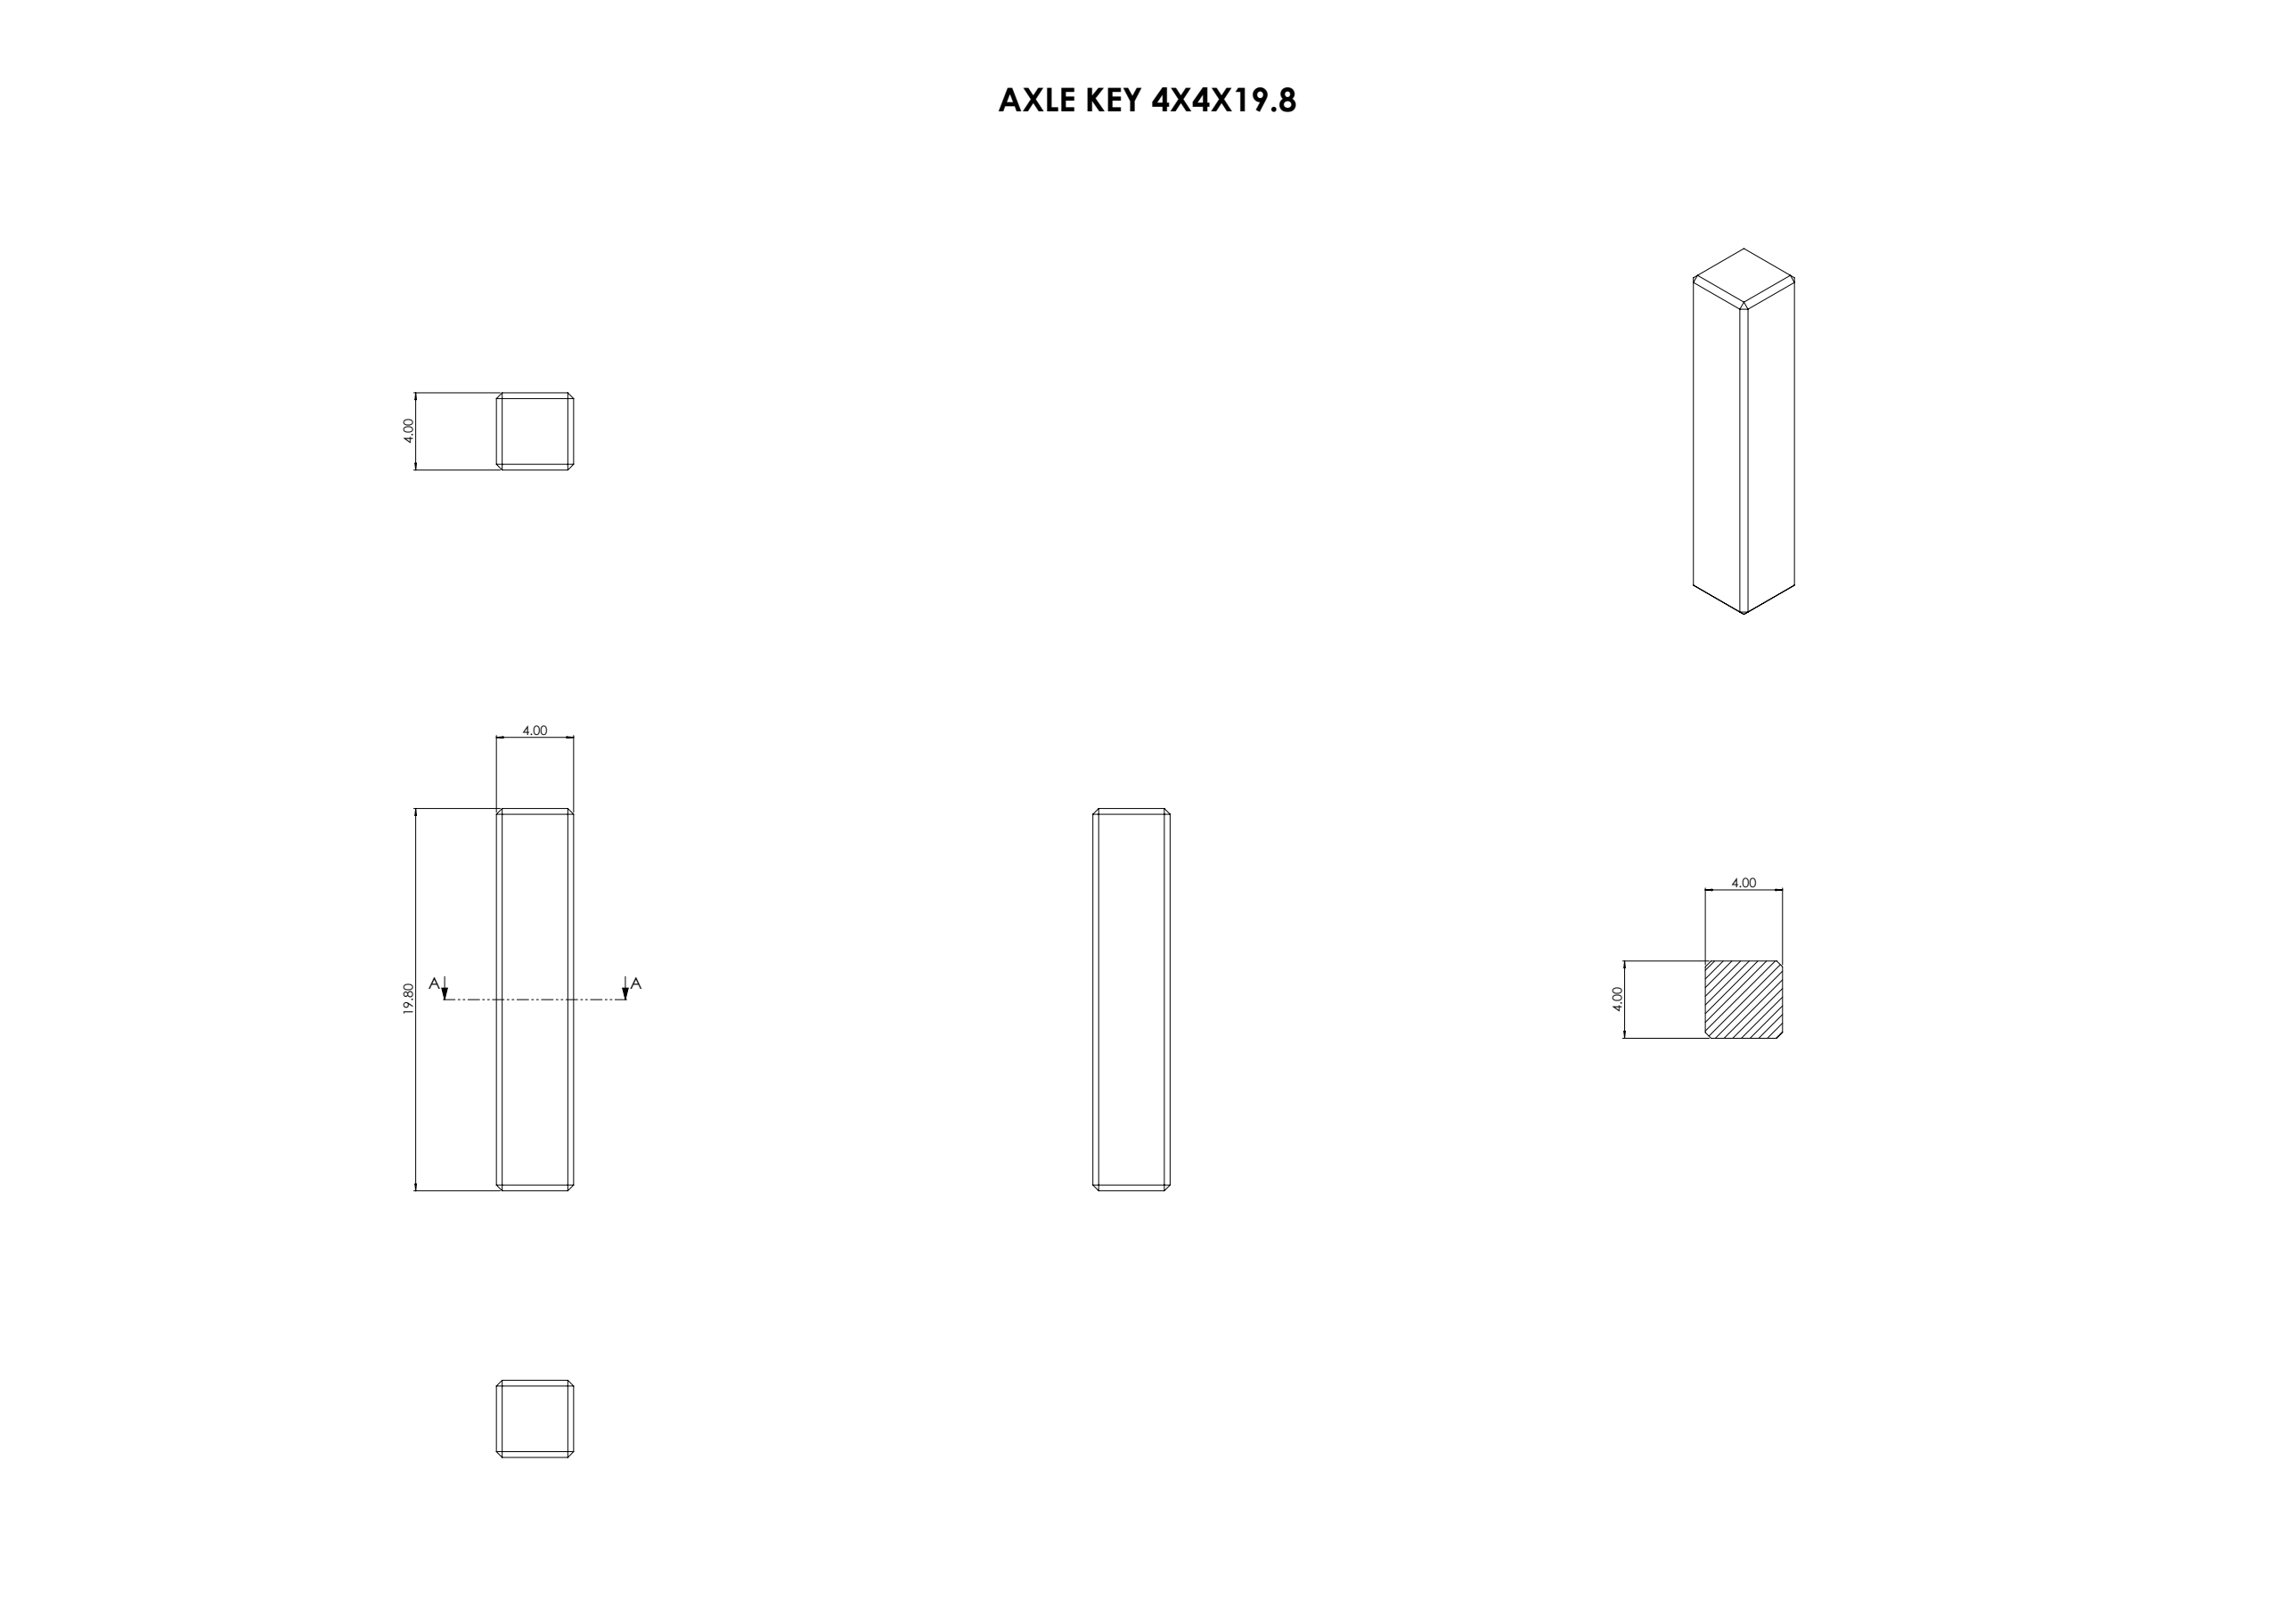
ISO-10303-21;
HEADER;
/* Generated by software containing ST-Developer
 * from STEP Tools, Inc. (www.steptools.com) 
 */

FILE_DESCRIPTION(
/* description */ (''),
/* implementation_level */ '2;1');

FILE_NAME(
/* name */ '09_Axle_Key_4x4x19.8.step',
/* time_stamp */ '2026-10-11T13:00:10-07:00',
/* author */ (''),
/* organization */ (''),
/* preprocessor_version */ 'ST-DEVELOPER v20.2',
/* originating_system */ 'Autodesk Translation Framework v15.15.0.0',
/* authorisation */ '');

FILE_SCHEMA (('AUTOMOTIVE_DESIGN { 1 0 10303 214 3 1 1 }'));
ENDSEC;

DATA;
#10=MECHANICAL_DESIGN_GEOMETRIC_PRESENTATION_REPRESENTATION('',(#366),#65563);
#344=SHAPE_REPRESENTATION_RELATIONSHIP('SRR','None',#65622,#355);
#355=ADVANCED_BREP_SHAPE_REPRESENTATION('',(#377),#65560);
#366=STYLED_ITEM('',(#65788),#377);
#377=MANIFOLD_SOLID_BREP('Body1',#20016);
#1012=PLANE('',#22010);
#1013=PLANE('',#22011);
#1014=PLANE('',#22012);
#1015=PLANE('',#22013);
#1016=PLANE('',#22014);
#1017=PLANE('',#22015);
#1018=PLANE('',#22016);
#1019=PLANE('',#22017);
#1020=PLANE('',#22018);
#1021=PLANE('',#22019);
#1022=PLANE('',#22020);
#1023=PLANE('',#22021);
#1024=PLANE('',#22022);
#1025=PLANE('',#22023);
#1026=PLANE('',#22024);
#1027=PLANE('',#22025);
#1028=PLANE('',#22026);
#1029=PLANE('',#22027);
#1030=PLANE('',#22028);
#1031=PLANE('',#22029);
#1032=PLANE('',#22030);
#1033=PLANE('',#22031);
#1034=PLANE('',#22032);
#1035=PLANE('',#22033);
#1036=PLANE('',#22034);
#1037=PLANE('',#22035);
#2122=FACE_OUTER_BOUND('',#3350,.T.);
#2123=FACE_OUTER_BOUND('',#3351,.T.);
#2124=FACE_OUTER_BOUND('',#3352,.T.);
#2125=FACE_OUTER_BOUND('',#3353,.T.);
#2126=FACE_OUTER_BOUND('',#3354,.T.);
#2127=FACE_OUTER_BOUND('',#3355,.T.);
#2128=FACE_OUTER_BOUND('',#3356,.T.);
#2129=FACE_OUTER_BOUND('',#3357,.T.);
#2130=FACE_OUTER_BOUND('',#3358,.T.);
#2131=FACE_OUTER_BOUND('',#3359,.T.);
#2132=FACE_OUTER_BOUND('',#3360,.T.);
#2133=FACE_OUTER_BOUND('',#3361,.T.);
#2134=FACE_OUTER_BOUND('',#3362,.T.);
#2135=FACE_OUTER_BOUND('',#3363,.T.);
#2136=FACE_OUTER_BOUND('',#3364,.T.);
#2137=FACE_OUTER_BOUND('',#3365,.T.);
#2138=FACE_OUTER_BOUND('',#3366,.T.);
#2139=FACE_OUTER_BOUND('',#3367,.T.);
#2140=FACE_OUTER_BOUND('',#3368,.T.);
#2141=FACE_OUTER_BOUND('',#3369,.T.);
#2142=FACE_OUTER_BOUND('',#3370,.T.);
#2143=FACE_OUTER_BOUND('',#3371,.T.);
#2144=FACE_OUTER_BOUND('',#3372,.T.);
#2145=FACE_OUTER_BOUND('',#3373,.T.);
#2146=FACE_OUTER_BOUND('',#3374,.T.);
#2147=FACE_OUTER_BOUND('',#3375,.T.);
#3350=EDGE_LOOP('',(#17338,#17339,#17340));
#3351=EDGE_LOOP('',(#17341,#17342,#17343));
#3352=EDGE_LOOP('',(#17344,#17345,#17346));
#3353=EDGE_LOOP('',(#17347,#17348,#17349));
#3354=EDGE_LOOP('',(#17350,#17351,#17352,#17353));
#3355=EDGE_LOOP('',(#17354,#17355,#17356));
#3356=EDGE_LOOP('',(#17357,#17358,#17359));
#3357=EDGE_LOOP('',(#17360,#17361,#17362,#17363));
#3358=EDGE_LOOP('',(#17364,#17365,#17366));
#3359=EDGE_LOOP('',(#17367,#17368,#17369,#17370));
#3360=EDGE_LOOP('',(#17371,#17372,#17373,#17374));
#3361=EDGE_LOOP('',(#17375,#17376,#17377));
#3362=EDGE_LOOP('',(#17378,#17379,#17380,#17381));
#3363=EDGE_LOOP('',(#17382,#17383,#17384,#17385));
#3364=EDGE_LOOP('',(#17386,#17387,#17388,#17389));
#3365=EDGE_LOOP('',(#17390,#17391,#17392,#17393));
#3366=EDGE_LOOP('',(#17394,#17395,#17396,#17397));
#3367=EDGE_LOOP('',(#17398,#17399,#17400,#17401));
#3368=EDGE_LOOP('',(#17402,#17403,#17404,#17405));
#3369=EDGE_LOOP('',(#17406,#17407,#17408,#17409));
#3370=EDGE_LOOP('',(#17410,#17411,#17412,#17413));
#3371=EDGE_LOOP('',(#17414,#17415,#17416,#17417));
#3372=EDGE_LOOP('',(#17418,#17419,#17420,#17421));
#3373=EDGE_LOOP('',(#17422,#17423,#17424,#17425));
#3374=EDGE_LOOP('',(#17426,#17427,#17428,#17429));
#3375=EDGE_LOOP('',(#17430,#17431,#17432,#17433));
#6130=LINE('',#62589,#7022);
#6131=LINE('',#62591,#7023);
#6132=LINE('',#62592,#7024);
#6133=LINE('',#62596,#7025);
#6134=LINE('',#62598,#7026);
#6135=LINE('',#62599,#7027);
#6136=LINE('',#62603,#7028);
#6137=LINE('',#62605,#7029);
#6138=LINE('',#62606,#7030);
#6139=LINE('',#62610,#7031);
#6140=LINE('',#62612,#7032);
#6141=LINE('',#62613,#7033);
#6142=LINE('',#62615,#7034);
#6143=LINE('',#62616,#7035);
#6144=LINE('',#62620,#7036);
#6145=LINE('',#62622,#7037);
#6146=LINE('',#62623,#7038);
#6147=LINE('',#62627,#7039);
#6148=LINE('',#62629,#7040);
#6149=LINE('',#62630,#7041);
#6150=LINE('',#62632,#7042);
#6151=LINE('',#62633,#7043);
#6152=LINE('',#62637,#7044);
#6153=LINE('',#62639,#7045);
#6154=LINE('',#62640,#7046);
#6155=LINE('',#62642,#7047);
#6156=LINE('',#62643,#7048);
#6157=LINE('',#62645,#7049);
#6158=LINE('',#62646,#7050);
#6159=LINE('',#62650,#7051);
#6160=LINE('',#62652,#7052);
#6161=LINE('',#62653,#7053);
#6162=LINE('',#62655,#7054);
#6163=LINE('',#62656,#7055);
#6164=LINE('',#62658,#7056);
#6165=LINE('',#62659,#7057);
#6166=LINE('',#62661,#7058);
#6167=LINE('',#62662,#7059);
#6168=LINE('',#62664,#7060);
#6169=LINE('',#62665,#7061);
#6170=LINE('',#62667,#7062);
#6171=LINE('',#62668,#7063);
#6172=LINE('',#62670,#7064);
#6173=LINE('',#62671,#7065);
#6174=LINE('',#62673,#7066);
#6175=LINE('',#62674,#7067);
#6176=LINE('',#62676,#7068);
#6177=LINE('',#62677,#7069);
#7022=VECTOR('',#26831,10.);
#7023=VECTOR('',#26832,10.);
#7024=VECTOR('',#26833,10.);
#7025=VECTOR('',#26836,10.);
#7026=VECTOR('',#26837,10.);
#7027=VECTOR('',#26838,10.);
#7028=VECTOR('',#26841,10.);
#7029=VECTOR('',#26842,10.);
#7030=VECTOR('',#26843,10.);
#7031=VECTOR('',#26846,10.);
#7032=VECTOR('',#26847,10.);
#7033=VECTOR('',#26848,10.);
#7034=VECTOR('',#26851,10.);
#7035=VECTOR('',#26852,10.);
#7036=VECTOR('',#26855,10.);
#7037=VECTOR('',#26856,10.);
#7038=VECTOR('',#26857,10.);
#7039=VECTOR('',#26860,10.);
#7040=VECTOR('',#26861,10.);
#7041=VECTOR('',#26862,10.);
#7042=VECTOR('',#26865,10.);
#7043=VECTOR('',#26866,10.);
#7044=VECTOR('',#26869,10.);
#7045=VECTOR('',#26870,10.);
#7046=VECTOR('',#26871,10.);
#7047=VECTOR('',#26874,10.);
#7048=VECTOR('',#26875,10.);
#7049=VECTOR('',#26878,10.);
#7050=VECTOR('',#26879,10.);
#7051=VECTOR('',#26882,10.);
#7052=VECTOR('',#26883,10.);
#7053=VECTOR('',#26884,10.);
#7054=VECTOR('',#26887,10.);
#7055=VECTOR('',#26888,10.);
#7056=VECTOR('',#26891,10.);
#7057=VECTOR('',#26892,10.);
#7058=VECTOR('',#26895,10.);
#7059=VECTOR('',#26896,10.);
#7060=VECTOR('',#26899,10.);
#7061=VECTOR('',#26900,10.);
#7062=VECTOR('',#26903,10.);
#7063=VECTOR('',#26904,10.);
#7064=VECTOR('',#26907,10.);
#7065=VECTOR('',#26908,10.);
#7066=VECTOR('',#26911,10.);
#7067=VECTOR('',#26912,10.);
#7068=VECTOR('',#26915,10.);
#7069=VECTOR('',#26916,10.);
#8833=VERTEX_POINT('',#62587);
#8834=VERTEX_POINT('',#62588);
#8835=VERTEX_POINT('',#62590);
#8836=VERTEX_POINT('',#62594);
#8837=VERTEX_POINT('',#62595);
#8838=VERTEX_POINT('',#62597);
#8839=VERTEX_POINT('',#62601);
#8840=VERTEX_POINT('',#62602);
#8841=VERTEX_POINT('',#62604);
#8842=VERTEX_POINT('',#62608);
#8843=VERTEX_POINT('',#62609);
#8844=VERTEX_POINT('',#62611);
#8845=VERTEX_POINT('',#62618);
#8846=VERTEX_POINT('',#62619);
#8847=VERTEX_POINT('',#62621);
#8848=VERTEX_POINT('',#62625);
#8849=VERTEX_POINT('',#62626);
#8850=VERTEX_POINT('',#62628);
#8851=VERTEX_POINT('',#62635);
#8852=VERTEX_POINT('',#62636);
#8853=VERTEX_POINT('',#62638);
#8854=VERTEX_POINT('',#62648);
#8855=VERTEX_POINT('',#62649);
#8856=VERTEX_POINT('',#62651);
#11702=EDGE_CURVE('',#8833,#8834,#6130,.T.);
#11703=EDGE_CURVE('',#8835,#8833,#6131,.T.);
#11704=EDGE_CURVE('',#8834,#8835,#6132,.T.);
#11705=EDGE_CURVE('',#8836,#8837,#6133,.T.);
#11706=EDGE_CURVE('',#8838,#8836,#6134,.T.);
#11707=EDGE_CURVE('',#8837,#8838,#6135,.T.);
#11708=EDGE_CURVE('',#8839,#8840,#6136,.T.);
#11709=EDGE_CURVE('',#8841,#8839,#6137,.T.);
#11710=EDGE_CURVE('',#8840,#8841,#6138,.T.);
#11711=EDGE_CURVE('',#8842,#8843,#6139,.T.);
#11712=EDGE_CURVE('',#8844,#8842,#6140,.T.);
#11713=EDGE_CURVE('',#8843,#8844,#6141,.T.);
#11714=EDGE_CURVE('',#8833,#8844,#6142,.T.);
#11715=EDGE_CURVE('',#8842,#8835,#6143,.T.);
#11716=EDGE_CURVE('',#8845,#8846,#6144,.T.);
#11717=EDGE_CURVE('',#8847,#8845,#6145,.T.);
#11718=EDGE_CURVE('',#8846,#8847,#6146,.T.);
#11719=EDGE_CURVE('',#8848,#8849,#6147,.T.);
#11720=EDGE_CURVE('',#8850,#8848,#6148,.T.);
#11721=EDGE_CURVE('',#8849,#8850,#6149,.T.);
#11722=EDGE_CURVE('',#8836,#8850,#6150,.T.);
#11723=EDGE_CURVE('',#8848,#8838,#6151,.T.);
#11724=EDGE_CURVE('',#8851,#8852,#6152,.T.);
#11725=EDGE_CURVE('',#8853,#8851,#6153,.T.);
#11726=EDGE_CURVE('',#8852,#8853,#6154,.T.);
#11727=EDGE_CURVE('',#8851,#8841,#6155,.T.);
#11728=EDGE_CURVE('',#8839,#8853,#6156,.T.);
#11729=EDGE_CURVE('',#8843,#8852,#6157,.T.);
#11730=EDGE_CURVE('',#8853,#8842,#6158,.T.);
#11731=EDGE_CURVE('',#8854,#8855,#6159,.T.);
#11732=EDGE_CURVE('',#8856,#8854,#6160,.T.);
#11733=EDGE_CURVE('',#8855,#8856,#6161,.T.);
#11734=EDGE_CURVE('',#8845,#8856,#6162,.T.);
#11735=EDGE_CURVE('',#8854,#8847,#6163,.T.);
#11736=EDGE_CURVE('',#8852,#8855,#6164,.T.);
#11737=EDGE_CURVE('',#8856,#8851,#6165,.T.);
#11738=EDGE_CURVE('',#8855,#8849,#6166,.T.);
#11739=EDGE_CURVE('',#8850,#8854,#6167,.T.);
#11740=EDGE_CURVE('',#8849,#8843,#6168,.T.);
#11741=EDGE_CURVE('',#8844,#8848,#6169,.T.);
#11742=EDGE_CURVE('',#8837,#8846,#6170,.T.);
#11743=EDGE_CURVE('',#8847,#8836,#6171,.T.);
#11744=EDGE_CURVE('',#8846,#8840,#6172,.T.);
#11745=EDGE_CURVE('',#8841,#8845,#6173,.T.);
#11746=EDGE_CURVE('',#8840,#8834,#6174,.T.);
#11747=EDGE_CURVE('',#8835,#8839,#6175,.T.);
#11748=EDGE_CURVE('',#8834,#8837,#6176,.T.);
#11749=EDGE_CURVE('',#8838,#8833,#6177,.T.);
#17338=ORIENTED_EDGE('',*,*,#11702,.F.);
#17339=ORIENTED_EDGE('',*,*,#11703,.F.);
#17340=ORIENTED_EDGE('',*,*,#11704,.F.);
#17341=ORIENTED_EDGE('',*,*,#11705,.F.);
#17342=ORIENTED_EDGE('',*,*,#11706,.F.);
#17343=ORIENTED_EDGE('',*,*,#11707,.F.);
#17344=ORIENTED_EDGE('',*,*,#11708,.F.);
#17345=ORIENTED_EDGE('',*,*,#11709,.F.);
#17346=ORIENTED_EDGE('',*,*,#11710,.F.);
#17347=ORIENTED_EDGE('',*,*,#11711,.F.);
#17348=ORIENTED_EDGE('',*,*,#11712,.F.);
#17349=ORIENTED_EDGE('',*,*,#11713,.F.);
#17350=ORIENTED_EDGE('',*,*,#11703,.T.);
#17351=ORIENTED_EDGE('',*,*,#11714,.T.);
#17352=ORIENTED_EDGE('',*,*,#11712,.T.);
#17353=ORIENTED_EDGE('',*,*,#11715,.T.);
#17354=ORIENTED_EDGE('',*,*,#11716,.F.);
#17355=ORIENTED_EDGE('',*,*,#11717,.F.);
#17356=ORIENTED_EDGE('',*,*,#11718,.F.);
#17357=ORIENTED_EDGE('',*,*,#11719,.F.);
#17358=ORIENTED_EDGE('',*,*,#11720,.F.);
#17359=ORIENTED_EDGE('',*,*,#11721,.F.);
#17360=ORIENTED_EDGE('',*,*,#11706,.T.);
#17361=ORIENTED_EDGE('',*,*,#11722,.T.);
#17362=ORIENTED_EDGE('',*,*,#11720,.T.);
#17363=ORIENTED_EDGE('',*,*,#11723,.T.);
#17364=ORIENTED_EDGE('',*,*,#11724,.F.);
#17365=ORIENTED_EDGE('',*,*,#11725,.F.);
#17366=ORIENTED_EDGE('',*,*,#11726,.F.);
#17367=ORIENTED_EDGE('',*,*,#11725,.T.);
#17368=ORIENTED_EDGE('',*,*,#11727,.T.);
#17369=ORIENTED_EDGE('',*,*,#11709,.T.);
#17370=ORIENTED_EDGE('',*,*,#11728,.T.);
#17371=ORIENTED_EDGE('',*,*,#11711,.T.);
#17372=ORIENTED_EDGE('',*,*,#11729,.T.);
#17373=ORIENTED_EDGE('',*,*,#11726,.T.);
#17374=ORIENTED_EDGE('',*,*,#11730,.T.);
#17375=ORIENTED_EDGE('',*,*,#11731,.F.);
#17376=ORIENTED_EDGE('',*,*,#11732,.F.);
#17377=ORIENTED_EDGE('',*,*,#11733,.F.);
#17378=ORIENTED_EDGE('',*,*,#11717,.T.);
#17379=ORIENTED_EDGE('',*,*,#11734,.T.);
#17380=ORIENTED_EDGE('',*,*,#11732,.T.);
#17381=ORIENTED_EDGE('',*,*,#11735,.T.);
#17382=ORIENTED_EDGE('',*,*,#11724,.T.);
#17383=ORIENTED_EDGE('',*,*,#11736,.T.);
#17384=ORIENTED_EDGE('',*,*,#11733,.T.);
#17385=ORIENTED_EDGE('',*,*,#11737,.T.);
#17386=ORIENTED_EDGE('',*,*,#11731,.T.);
#17387=ORIENTED_EDGE('',*,*,#11738,.T.);
#17388=ORIENTED_EDGE('',*,*,#11721,.T.);
#17389=ORIENTED_EDGE('',*,*,#11739,.T.);
#17390=ORIENTED_EDGE('',*,*,#11719,.T.);
#17391=ORIENTED_EDGE('',*,*,#11740,.T.);
#17392=ORIENTED_EDGE('',*,*,#11713,.T.);
#17393=ORIENTED_EDGE('',*,*,#11741,.T.);
#17394=ORIENTED_EDGE('',*,*,#11705,.T.);
#17395=ORIENTED_EDGE('',*,*,#11742,.T.);
#17396=ORIENTED_EDGE('',*,*,#11718,.T.);
#17397=ORIENTED_EDGE('',*,*,#11743,.T.);
#17398=ORIENTED_EDGE('',*,*,#11716,.T.);
#17399=ORIENTED_EDGE('',*,*,#11744,.T.);
#17400=ORIENTED_EDGE('',*,*,#11710,.T.);
#17401=ORIENTED_EDGE('',*,*,#11745,.T.);
#17402=ORIENTED_EDGE('',*,*,#11708,.T.);
#17403=ORIENTED_EDGE('',*,*,#11746,.T.);
#17404=ORIENTED_EDGE('',*,*,#11704,.T.);
#17405=ORIENTED_EDGE('',*,*,#11747,.T.);
#17406=ORIENTED_EDGE('',*,*,#11702,.T.);
#17407=ORIENTED_EDGE('',*,*,#11748,.T.);
#17408=ORIENTED_EDGE('',*,*,#11707,.T.);
#17409=ORIENTED_EDGE('',*,*,#11749,.T.);
#17410=ORIENTED_EDGE('',*,*,#11723,.F.);
#17411=ORIENTED_EDGE('',*,*,#11741,.F.);
#17412=ORIENTED_EDGE('',*,*,#11714,.F.);
#17413=ORIENTED_EDGE('',*,*,#11749,.F.);
#17414=ORIENTED_EDGE('',*,*,#11728,.F.);
#17415=ORIENTED_EDGE('',*,*,#11747,.F.);
#17416=ORIENTED_EDGE('',*,*,#11715,.F.);
#17417=ORIENTED_EDGE('',*,*,#11730,.F.);
#17418=ORIENTED_EDGE('',*,*,#11729,.F.);
#17419=ORIENTED_EDGE('',*,*,#11740,.F.);
#17420=ORIENTED_EDGE('',*,*,#11738,.F.);
#17421=ORIENTED_EDGE('',*,*,#11736,.F.);
#17422=ORIENTED_EDGE('',*,*,#11735,.F.);
#17423=ORIENTED_EDGE('',*,*,#11739,.F.);
#17424=ORIENTED_EDGE('',*,*,#11722,.F.);
#17425=ORIENTED_EDGE('',*,*,#11743,.F.);
#17426=ORIENTED_EDGE('',*,*,#11734,.F.);
#17427=ORIENTED_EDGE('',*,*,#11745,.F.);
#17428=ORIENTED_EDGE('',*,*,#11727,.F.);
#17429=ORIENTED_EDGE('',*,*,#11737,.F.);
#17430=ORIENTED_EDGE('',*,*,#11742,.F.);
#17431=ORIENTED_EDGE('',*,*,#11748,.F.);
#17432=ORIENTED_EDGE('',*,*,#11746,.F.);
#17433=ORIENTED_EDGE('',*,*,#11744,.F.);
#19818=ADVANCED_FACE('',(#2122),#1012,.T.);
#19819=ADVANCED_FACE('',(#2123),#1013,.T.);
#19820=ADVANCED_FACE('',(#2124),#1014,.T.);
#19821=ADVANCED_FACE('',(#2125),#1015,.T.);
#19822=ADVANCED_FACE('',(#2126),#1016,.T.);
#19823=ADVANCED_FACE('',(#2127),#1017,.T.);
#19824=ADVANCED_FACE('',(#2128),#1018,.T.);
#19825=ADVANCED_FACE('',(#2129),#1019,.T.);
#19826=ADVANCED_FACE('',(#2130),#1020,.T.);
#19827=ADVANCED_FACE('',(#2131),#1021,.T.);
#19828=ADVANCED_FACE('',(#2132),#1022,.T.);
#19829=ADVANCED_FACE('',(#2133),#1023,.T.);
#19830=ADVANCED_FACE('',(#2134),#1024,.T.);
#19831=ADVANCED_FACE('',(#2135),#1025,.T.);
#19832=ADVANCED_FACE('',(#2136),#1026,.T.);
#19833=ADVANCED_FACE('',(#2137),#1027,.T.);
#19834=ADVANCED_FACE('',(#2138),#1028,.T.);
#19835=ADVANCED_FACE('',(#2139),#1029,.T.);
#19836=ADVANCED_FACE('',(#2140),#1030,.T.);
#19837=ADVANCED_FACE('',(#2141),#1031,.T.);
#19838=ADVANCED_FACE('',(#2142),#1032,.T.);
#19839=ADVANCED_FACE('',(#2143),#1033,.T.);
#19840=ADVANCED_FACE('',(#2144),#1034,.T.);
#19841=ADVANCED_FACE('',(#2145),#1035,.T.);
#19842=ADVANCED_FACE('',(#2146),#1036,.T.);
#19843=ADVANCED_FACE('',(#2147),#1037,.T.);
#20016=CLOSED_SHELL('',(#19818,#19819,#19820,#19821,#19822,#19823,#19824,
#19825,#19826,#19827,#19828,#19829,#19830,#19831,#19832,#19833,#19834,#19835,
#19836,#19837,#19838,#19839,#19840,#19841,#19842,#19843));
#22009=AXIS2_PLACEMENT_3D('',#62585,#26827,#26828);
#22010=AXIS2_PLACEMENT_3D('',#62586,#26829,#26830);
#22011=AXIS2_PLACEMENT_3D('',#62593,#26834,#26835);
#22012=AXIS2_PLACEMENT_3D('',#62600,#26839,#26840);
#22013=AXIS2_PLACEMENT_3D('',#62607,#26844,#26845);
#22014=AXIS2_PLACEMENT_3D('',#62614,#26849,#26850);
#22015=AXIS2_PLACEMENT_3D('',#62617,#26853,#26854);
#22016=AXIS2_PLACEMENT_3D('',#62624,#26858,#26859);
#22017=AXIS2_PLACEMENT_3D('',#62631,#26863,#26864);
#22018=AXIS2_PLACEMENT_3D('',#62634,#26867,#26868);
#22019=AXIS2_PLACEMENT_3D('',#62641,#26872,#26873);
#22020=AXIS2_PLACEMENT_3D('',#62644,#26876,#26877);
#22021=AXIS2_PLACEMENT_3D('',#62647,#26880,#26881);
#22022=AXIS2_PLACEMENT_3D('',#62654,#26885,#26886);
#22023=AXIS2_PLACEMENT_3D('',#62657,#26889,#26890);
#22024=AXIS2_PLACEMENT_3D('',#62660,#26893,#26894);
#22025=AXIS2_PLACEMENT_3D('',#62663,#26897,#26898);
#22026=AXIS2_PLACEMENT_3D('',#62666,#26901,#26902);
#22027=AXIS2_PLACEMENT_3D('',#62669,#26905,#26906);
#22028=AXIS2_PLACEMENT_3D('',#62672,#26909,#26910);
#22029=AXIS2_PLACEMENT_3D('',#62675,#26913,#26914);
#22030=AXIS2_PLACEMENT_3D('',#62678,#26917,#26918);
#22031=AXIS2_PLACEMENT_3D('',#62679,#26919,#26920);
#22032=AXIS2_PLACEMENT_3D('',#62680,#26921,#26922);
#22033=AXIS2_PLACEMENT_3D('',#62681,#26923,#26924);
#22034=AXIS2_PLACEMENT_3D('',#62682,#26925,#26926);
#22035=AXIS2_PLACEMENT_3D('',#62683,#26927,#26928);
#26827=DIRECTION('axis',(0.,0.,1.));
#26828=DIRECTION('refdir',(1.,0.,0.));
#26829=DIRECTION('center_axis',(0.577350269189626,0.577350269189626,0.577350269189626));
#26830=DIRECTION('ref_axis',(0.707106781186548,0.,-0.707106781186547));
#26831=DIRECTION('',(-0.707106781186548,0.,0.707106781186547));
#26832=DIRECTION('',(0.707106781186548,-0.707106781186548,0.));
#26833=DIRECTION('',(0.,0.707106781186548,-0.707106781186547));
#26834=DIRECTION('center_axis',(0.577350269189626,-0.577350269189626,0.577350269189626));
#26835=DIRECTION('ref_axis',(0.707106781186548,0.,-0.707106781186547));
#26836=DIRECTION('',(0.,0.707106781186548,0.707106781186547));
#26837=DIRECTION('',(-0.707106781186548,-0.707106781186548,0.));
#26838=DIRECTION('',(0.707106781186548,0.,-0.707106781186547));
#26839=DIRECTION('center_axis',(-0.577350269189626,0.577350269189626,0.577350269189626));
#26840=DIRECTION('ref_axis',(0.707106781186548,0.,0.707106781186547));
#26841=DIRECTION('',(0.,-0.707106781186548,0.707106781186547));
#26842=DIRECTION('',(0.707106781186548,0.707106781186548,0.));
#26843=DIRECTION('',(-0.707106781186548,0.,-0.707106781186547));
#26844=DIRECTION('center_axis',(0.577350269189626,0.577350269189626,-0.577350269189626));
#26845=DIRECTION('ref_axis',(-0.707106781186548,0.,-0.707106781186547));
#26846=DIRECTION('',(0.,-0.707106781186548,-0.707106781186547));
#26847=DIRECTION('',(-0.707106781186548,0.707106781186548,0.));
#26848=DIRECTION('',(0.707106781186548,0.,0.707106781186547));
#26849=DIRECTION('center_axis',(0.707106781186548,0.707106781186548,0.));
#26850=DIRECTION('ref_axis',(0.,0.,-1.));
#26851=DIRECTION('',(0.,0.,-1.));
#26852=DIRECTION('',(0.,0.,1.));
#26853=DIRECTION('center_axis',(-0.577350269189624,-0.577350269189629,0.577350269189625));
#26854=DIRECTION('ref_axis',(0.707106781186548,0.,0.707106781186547));
#26855=DIRECTION('',(0.707106781186548,0.,0.707106781186547));
#26856=DIRECTION('',(-0.70710678118655,0.707106781186545,0.));
#26857=DIRECTION('',(5.23364152894591E-15,-0.707106781186548,-0.707106781186547));
#26858=DIRECTION('center_axis',(0.577350269189626,-0.577350269189626,-0.577350269189626));
#26859=DIRECTION('ref_axis',(-0.707106781186548,0.,-0.707106781186547));
#26860=DIRECTION('',(-0.707106781186548,0.,-0.707106781186547));
#26861=DIRECTION('',(0.707106781186548,0.707106781186548,0.));
#26862=DIRECTION('',(0.,-0.707106781186548,0.707106781186547));
#26863=DIRECTION('center_axis',(0.707106781186548,-0.707106781186548,0.));
#26864=DIRECTION('ref_axis',(0.,0.,-1.));
#26865=DIRECTION('',(0.,0.,-1.));
#26866=DIRECTION('',(0.,0.,1.));
#26867=DIRECTION('center_axis',(-0.577350269189626,0.577350269189626,-0.577350269189626));
#26868=DIRECTION('ref_axis',(-0.707106781186548,0.,0.707106781186547));
#26869=DIRECTION('',(0.707106781186548,0.,-0.707106781186547));
#26870=DIRECTION('',(-0.707106781186548,-0.707106781186548,0.));
#26871=DIRECTION('',(0.,0.707106781186548,0.707106781186547));
#26872=DIRECTION('center_axis',(-0.707106781186548,0.707106781186548,0.));
#26873=DIRECTION('ref_axis',(0.,0.,1.));
#26874=DIRECTION('',(0.,0.,1.));
#26875=DIRECTION('',(0.,0.,-1.));
#26876=DIRECTION('center_axis',(0.,0.707106781186547,-0.707106781186548));
#26877=DIRECTION('ref_axis',(-1.,0.,0.));
#26878=DIRECTION('',(-1.,0.,0.));
#26879=DIRECTION('',(1.,0.,0.));
#26880=DIRECTION('center_axis',(-0.577350269189624,-0.577350269189628,-0.577350269189625));
#26881=DIRECTION('ref_axis',(-0.707106781186548,0.,0.707106781186547));
#26882=DIRECTION('',(-5.23364152894591E-15,0.707106781186548,-0.707106781186547));
#26883=DIRECTION('',(0.70710678118655,-0.707106781186545,0.));
#26884=DIRECTION('',(-0.707106781186548,0.,0.707106781186547));
#26885=DIRECTION('center_axis',(-0.707106781186545,-0.70710678118655,0.));
#26886=DIRECTION('ref_axis',(0.,0.,1.));
#26887=DIRECTION('',(0.,0.,-1.));
#26888=DIRECTION('',(0.,0.,1.));
#26889=DIRECTION('center_axis',(-0.707106781186547,0.,-0.707106781186548));
#26890=DIRECTION('ref_axis',(-0.707106781186548,0.,0.707106781186547));
#26891=DIRECTION('',(0.,-1.,0.));
#26892=DIRECTION('',(0.,1.,0.));
#26893=DIRECTION('center_axis',(0.,-0.707106781186547,-0.707106781186548));
#26894=DIRECTION('ref_axis',(-1.,0.,0.));
#26895=DIRECTION('',(1.,0.,0.));
#26896=DIRECTION('',(-1.,0.,0.));
#26897=DIRECTION('center_axis',(0.707106781186547,0.,-0.707106781186548));
#26898=DIRECTION('ref_axis',(-0.707106781186548,0.,-0.707106781186547));
#26899=DIRECTION('',(0.,1.,0.));
#26900=DIRECTION('',(0.,-1.,0.));
#26901=DIRECTION('center_axis',(0.,-0.707106781186547,0.707106781186548));
#26902=DIRECTION('ref_axis',(1.,0.,0.));
#26903=DIRECTION('',(-1.,0.,0.));
#26904=DIRECTION('',(1.,0.,0.));
#26905=DIRECTION('center_axis',(-0.707106781186547,0.,0.707106781186548));
#26906=DIRECTION('ref_axis',(0.707106781186548,0.,0.707106781186547));
#26907=DIRECTION('',(0.,1.,0.));
#26908=DIRECTION('',(0.,-1.,0.));
#26909=DIRECTION('center_axis',(0.,0.707106781186547,0.707106781186548));
#26910=DIRECTION('ref_axis',(1.,0.,0.));
#26911=DIRECTION('',(1.,0.,0.));
#26912=DIRECTION('',(-1.,0.,0.));
#26913=DIRECTION('center_axis',(0.707106781186547,0.,0.707106781186548));
#26914=DIRECTION('ref_axis',(0.707106781186548,0.,-0.707106781186547));
#26915=DIRECTION('',(0.,-1.,0.));
#26916=DIRECTION('',(0.,1.,0.));
#26917=DIRECTION('center_axis',(1.,0.,0.));
#26918=DIRECTION('ref_axis',(0.,1.,0.));
#26919=DIRECTION('center_axis',(0.,1.,0.));
#26920=DIRECTION('ref_axis',(-1.,0.,0.));
#26921=DIRECTION('center_axis',(0.,0.,-1.));
#26922=DIRECTION('ref_axis',(-1.,0.,0.));
#26923=DIRECTION('center_axis',(0.,-1.,0.));
#26924=DIRECTION('ref_axis',(1.,0.,0.));
#26925=DIRECTION('center_axis',(-1.,0.,0.));
#26926=DIRECTION('ref_axis',(0.,-1.,0.));
#26927=DIRECTION('center_axis',(0.,0.,1.));
#26928=DIRECTION('ref_axis',(1.,0.,0.));
#62585=CARTESIAN_POINT('',(0.,0.,0.));
#62586=CARTESIAN_POINT('Origin',(-7.8,9.9,1.7));
#62587=CARTESIAN_POINT('',(-7.5,9.6,1.7));
#62588=CARTESIAN_POINT('',(-7.8,9.6,2.));
#62589=CARTESIAN_POINT('',(-7.5,9.6,1.7));
#62590=CARTESIAN_POINT('',(-7.8,9.9,1.7));
#62591=CARTESIAN_POINT('',(-7.8,9.9,1.7));
#62592=CARTESIAN_POINT('',(-7.8,9.6,2.));
#62593=CARTESIAN_POINT('Origin',(-7.5,-9.6,1.7));
#62594=CARTESIAN_POINT('',(-7.8,-9.9,1.7));
#62595=CARTESIAN_POINT('',(-7.8,-9.6,2.));
#62596=CARTESIAN_POINT('',(-7.8,-9.9,1.7));
#62597=CARTESIAN_POINT('',(-7.5,-9.6,1.7));
#62598=CARTESIAN_POINT('',(-7.5,-9.6,1.7));
#62599=CARTESIAN_POINT('',(-7.8,-9.6,2.));
#62600=CARTESIAN_POINT('Origin',(-11.5,9.6,1.7));
#62601=CARTESIAN_POINT('',(-11.2,9.9,1.7));
#62602=CARTESIAN_POINT('',(-11.2,9.6,2.));
#62603=CARTESIAN_POINT('',(-11.2,9.9,1.7));
#62604=CARTESIAN_POINT('',(-11.5,9.6,1.7));
#62605=CARTESIAN_POINT('',(-11.5,9.6,1.7));
#62606=CARTESIAN_POINT('',(-11.2,9.6,2.));
#62607=CARTESIAN_POINT('Origin',(-7.5,9.6,-1.7));
#62608=CARTESIAN_POINT('',(-7.8,9.9,-1.7));
#62609=CARTESIAN_POINT('',(-7.8,9.6,-2.));
#62610=CARTESIAN_POINT('',(-7.8,9.9,-1.7));
#62611=CARTESIAN_POINT('',(-7.5,9.6,-1.7));
#62612=CARTESIAN_POINT('',(-7.5,9.6,-1.7));
#62613=CARTESIAN_POINT('',(-7.8,9.6,-2.));
#62614=CARTESIAN_POINT('Origin',(-7.65,9.75,0.));
#62615=CARTESIAN_POINT('',(-7.5,9.6,0.));
#62616=CARTESIAN_POINT('',(-7.8,9.9,0.));
#62617=CARTESIAN_POINT('Origin',(-11.2,-9.9,1.7));
#62618=CARTESIAN_POINT('',(-11.5,-9.6,1.7));
#62619=CARTESIAN_POINT('',(-11.2,-9.6,2.));
#62620=CARTESIAN_POINT('',(-11.5,-9.6,1.7));
#62621=CARTESIAN_POINT('',(-11.2,-9.9,1.7));
#62622=CARTESIAN_POINT('',(-11.2,-9.9,1.7));
#62623=CARTESIAN_POINT('',(-11.2,-9.6,2.));
#62624=CARTESIAN_POINT('Origin',(-7.8,-9.9,-1.7));
#62625=CARTESIAN_POINT('',(-7.5,-9.6,-1.7));
#62626=CARTESIAN_POINT('',(-7.8,-9.6,-2.));
#62627=CARTESIAN_POINT('',(-7.5,-9.6,-1.7));
#62628=CARTESIAN_POINT('',(-7.8,-9.9,-1.7));
#62629=CARTESIAN_POINT('',(-7.8,-9.9,-1.7));
#62630=CARTESIAN_POINT('',(-7.8,-9.6,-2.));
#62631=CARTESIAN_POINT('Origin',(-7.65,-9.75,0.));
#62632=CARTESIAN_POINT('',(-7.8,-9.9,0.));
#62633=CARTESIAN_POINT('',(-7.5,-9.6,0.));
#62634=CARTESIAN_POINT('Origin',(-11.2,9.9,-1.7));
#62635=CARTESIAN_POINT('',(-11.5,9.6,-1.7));
#62636=CARTESIAN_POINT('',(-11.2,9.6,-2.));
#62637=CARTESIAN_POINT('',(-11.5,9.6,-1.7));
#62638=CARTESIAN_POINT('',(-11.2,9.9,-1.7));
#62639=CARTESIAN_POINT('',(-11.2,9.9,-1.7));
#62640=CARTESIAN_POINT('',(-11.2,9.6,-2.));
#62641=CARTESIAN_POINT('Origin',(-11.35,9.75,0.));
#62642=CARTESIAN_POINT('',(-11.5,9.6,0.));
#62643=CARTESIAN_POINT('',(-11.2,9.9,0.));
#62644=CARTESIAN_POINT('Origin',(-8.5,9.75,-1.85));
#62645=CARTESIAN_POINT('',(-8.5,9.6,-2.));
#62646=CARTESIAN_POINT('',(-8.5,9.9,-1.7));
#62647=CARTESIAN_POINT('Origin',(-11.5,-9.6,-1.7));
#62648=CARTESIAN_POINT('',(-11.2,-9.9,-1.7));
#62649=CARTESIAN_POINT('',(-11.2,-9.6,-2.));
#62650=CARTESIAN_POINT('',(-11.2,-9.9,-1.7));
#62651=CARTESIAN_POINT('',(-11.5,-9.6,-1.7));
#62652=CARTESIAN_POINT('',(-11.5,-9.6,-1.7));
#62653=CARTESIAN_POINT('',(-11.2,-9.6,-2.));
#62654=CARTESIAN_POINT('Origin',(-11.35,-9.75,0.));
#62655=CARTESIAN_POINT('',(-11.5,-9.6,0.));
#62656=CARTESIAN_POINT('',(-11.2,-9.9,0.));
#62657=CARTESIAN_POINT('Origin',(-11.35,4.95,-1.85));
#62658=CARTESIAN_POINT('',(-11.2,4.95,-2.));
#62659=CARTESIAN_POINT('',(-11.5,4.95,-1.7));
#62660=CARTESIAN_POINT('Origin',(-10.5,-9.75,-1.85));
#62661=CARTESIAN_POINT('',(-10.5,-9.6,-2.));
#62662=CARTESIAN_POINT('',(-10.5,-9.9,-1.7));
#62663=CARTESIAN_POINT('Origin',(-7.65,-4.95,-1.85));
#62664=CARTESIAN_POINT('',(-7.8,-4.95,-2.));
#62665=CARTESIAN_POINT('',(-7.5,-4.95,-1.7));
#62666=CARTESIAN_POINT('Origin',(-10.5,-9.75,1.85));
#62667=CARTESIAN_POINT('',(-10.5,-9.6,2.));
#62668=CARTESIAN_POINT('',(-10.5,-9.9,1.7));
#62669=CARTESIAN_POINT('Origin',(-11.35,4.95,1.85));
#62670=CARTESIAN_POINT('',(-11.2,4.95,2.));
#62671=CARTESIAN_POINT('',(-11.5,4.95,1.7));
#62672=CARTESIAN_POINT('Origin',(-8.5,9.75,1.85));
#62673=CARTESIAN_POINT('',(-8.5,9.6,2.));
#62674=CARTESIAN_POINT('',(-8.5,9.9,1.7));
#62675=CARTESIAN_POINT('Origin',(-7.65,-4.95,1.85));
#62676=CARTESIAN_POINT('',(-7.8,-4.95,2.));
#62677=CARTESIAN_POINT('',(-7.5,-4.95,1.7));
#62678=CARTESIAN_POINT('Origin',(-7.5,-9.9,0.));
#62679=CARTESIAN_POINT('Origin',(-7.5,9.9,0.));
#62680=CARTESIAN_POINT('Origin',(-9.5,0.,-2.));
#62681=CARTESIAN_POINT('Origin',(-11.5,-9.9,0.));
#62682=CARTESIAN_POINT('Origin',(-11.5,9.9,0.));
#62683=CARTESIAN_POINT('Origin',(-9.5,0.,2.));
#65547=UNCERTAINTY_MEASURE_WITH_UNIT(LENGTH_MEASURE(0.01),#65564,
'DISTANCE_ACCURACY_VALUE',
'Maximum model space distance between geometric entities at asserted c
onnectivities');
#65550=UNCERTAINTY_MEASURE_WITH_UNIT(LENGTH_MEASURE(0.01),#65564,
'DISTANCE_ACCURACY_VALUE',
'Maximum model space distance between geometric entities at asserted c
onnectivities');
#65560=(
GEOMETRIC_REPRESENTATION_CONTEXT(3)
GLOBAL_UNCERTAINTY_ASSIGNED_CONTEXT((#65547))
GLOBAL_UNIT_ASSIGNED_CONTEXT((#65564,#65566,#65567))
REPRESENTATION_CONTEXT('','3D')
);
#65563=(
GEOMETRIC_REPRESENTATION_CONTEXT(3)
GLOBAL_UNCERTAINTY_ASSIGNED_CONTEXT((#65550))
GLOBAL_UNIT_ASSIGNED_CONTEXT((#65564,#65566,#65567))
REPRESENTATION_CONTEXT('','3D')
);
#65564=(
LENGTH_UNIT()
NAMED_UNIT(*)
SI_UNIT(.MILLI.,.METRE.)
);
#65566=(
NAMED_UNIT(*)
PLANE_ANGLE_UNIT()
SI_UNIT($,.RADIAN.)
);
#65567=(
NAMED_UNIT(*)
SI_UNIT($,.STERADIAN.)
SOLID_ANGLE_UNIT()
);
#65577=SHAPE_DEFINITION_REPRESENTATION(#65589,#65622);
#65589=PRODUCT_DEFINITION_SHAPE('',$,#65635);
#65622=SHAPE_REPRESENTATION('',(#22009),#65560);
#65625=PRODUCT_DEFINITION_CONTEXT('part definition',#65663,'design');
#65635=PRODUCT_DEFINITION('2026-10-10-05-45-29-923',
'09_Axle_Key_4x4x19.8',#65647,#65625);
#65647=PRODUCT_DEFINITION_FORMATION('',$,#65674);
#65663=APPLICATION_CONTEXT(
'Core Data for Automotive Mechanical Design Process');
#65664=PRODUCT_CONTEXT('part definition',#65663,'mechanical');
#65674=PRODUCT('2026-10-10-05-45-29-923','09_Axle_Key_4x4x19.8',$,(#65664));
#65782=COLOUR_RGB('Grey',0.48,0.52,0.57);
#65783=FILL_AREA_STYLE_COLOUR('',#65782);
#65784=FILL_AREA_STYLE('',(#65783));
#65785=SURFACE_STYLE_FILL_AREA(#65784);
#65786=SURFACE_SIDE_STYLE('',(#65785));
#65787=SURFACE_STYLE_USAGE(.BOTH.,#65786);
#65788=PRESENTATION_STYLE_ASSIGNMENT((#65787));
ENDSEC;
END-ISO-10303-21;
